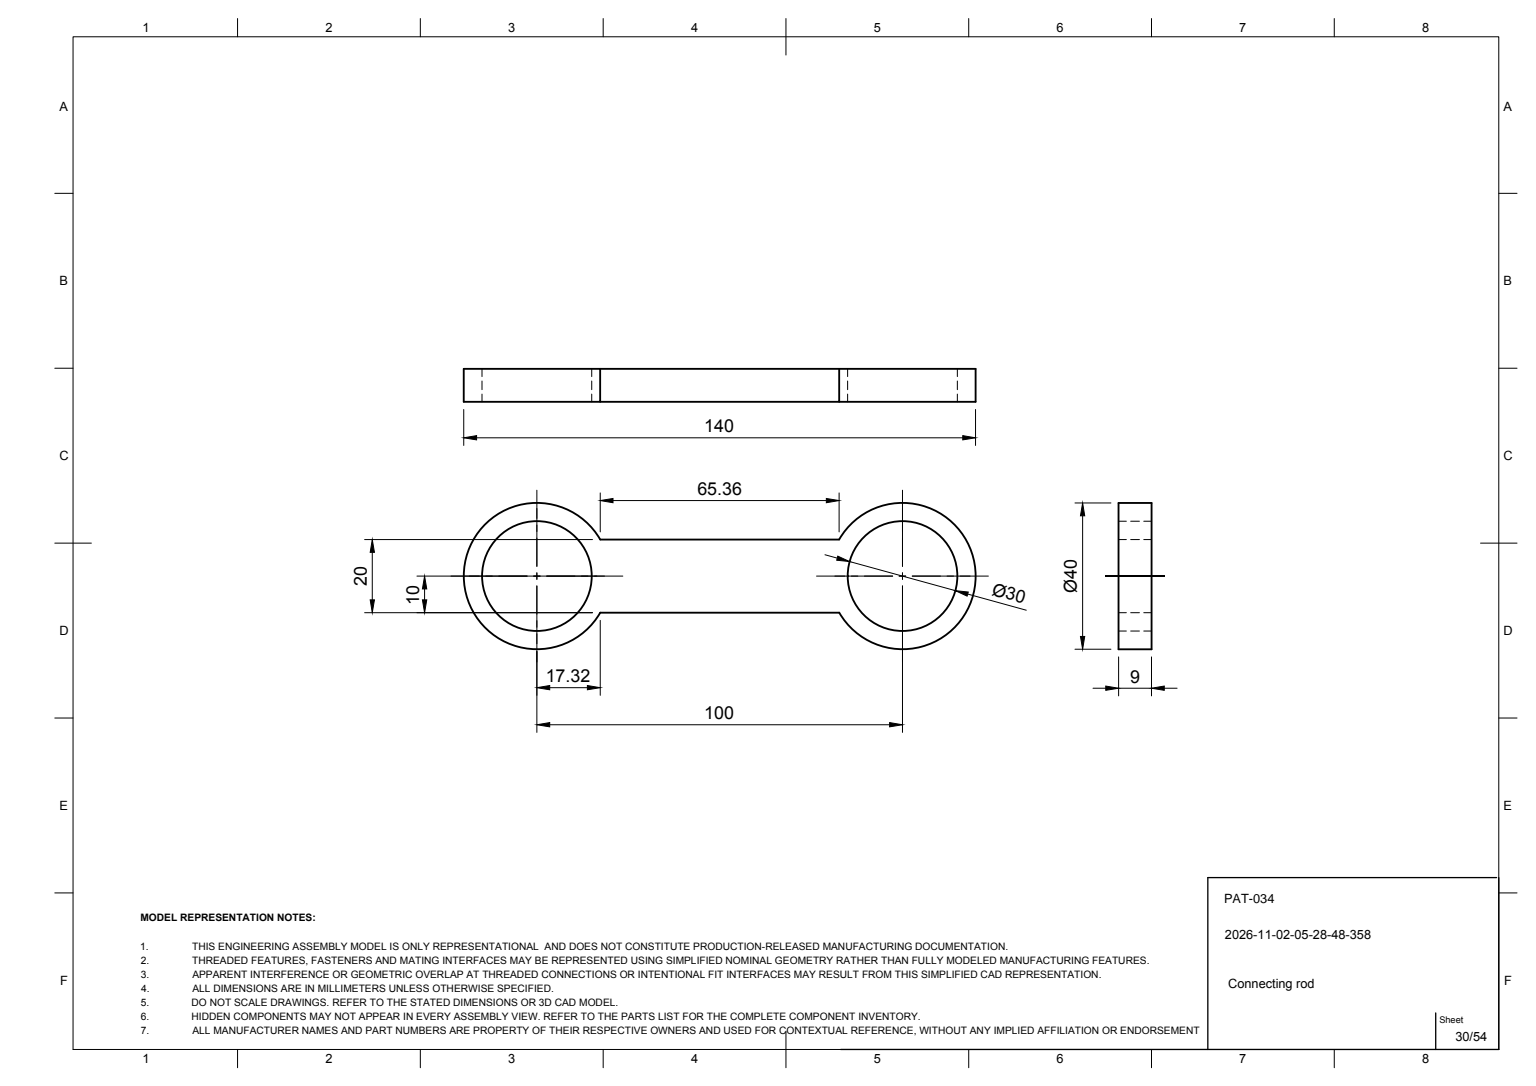
ISO-10303-21;
HEADER;
/* Generated by software containing ST-Developer
 * from STEP Tools, Inc. (www.steptools.com) 
 */

FILE_DESCRIPTION(
/* description */ ('Fatigue rig crank-slider'),
/* implementation_level */ '2;1');

FILE_NAME(
/* name */ 'Connecting rod.step',
/* time_stamp */ '2026-10-28T03:24:50-07:00',
/* author */ (''),
/* organization */ (''),
/* preprocessor_version */ 'ST-DEVELOPER v20.2',
/* originating_system */ 'Autodesk Translation Framework v15.17.0.0',
/* authorisation */ '');

FILE_SCHEMA (('AUTOMOTIVE_DESIGN { 1 0 10303 214 3 1 1 }'));
ENDSEC;

DATA;
#10=MECHANICAL_DESIGN_GEOMETRIC_PRESENTATION_REPRESENTATION('',(#615),#16911);
#514=SHAPE_REPRESENTATION_RELATIONSHIP('SRR','None',#17156,#564);
#564=ADVANCED_BREP_SHAPE_REPRESENTATION('',(#672),#16885);
#615=STYLED_ITEM('',(#17487),#672);
#672=MANIFOLD_SOLID_BREP('Body1',#8908);
#842=FACE_BOUND('',#2187,.T.);
#843=FACE_BOUND('',#2188,.T.);
#844=FACE_BOUND('',#2193,.T.);
#845=FACE_BOUND('',#2194,.T.);
#1082=PLANE('',#10063);
#1083=PLANE('',#10065);
#1084=PLANE('',#10068);
#1085=PLANE('',#10069);
#1518=FACE_OUTER_BOUND('',#2183,.T.);
#1519=FACE_OUTER_BOUND('',#2184,.T.);
#1520=FACE_OUTER_BOUND('',#2185,.T.);
#1521=FACE_OUTER_BOUND('',#2186,.T.);
#1522=FACE_OUTER_BOUND('',#2189,.T.);
#1523=FACE_OUTER_BOUND('',#2190,.T.);
#1524=FACE_OUTER_BOUND('',#2191,.T.);
#1525=FACE_OUTER_BOUND('',#2192,.T.);
#2183=EDGE_LOOP('',(#7256,#7257,#7258,#7259));
#2184=EDGE_LOOP('',(#7260,#7261,#7262,#7263));
#2185=EDGE_LOOP('',(#7264,#7265,#7266,#7267));
#2186=EDGE_LOOP('',(#7268,#7269,#7270,#7271));
#2187=EDGE_LOOP('',(#7272));
#2188=EDGE_LOOP('',(#7273));
#2189=EDGE_LOOP('',(#7274,#7275,#7276,#7277));
#2190=EDGE_LOOP('',(#7278,#7279,#7280,#7281));
#2191=EDGE_LOOP('',(#7282,#7283,#7284,#7285));
#2192=EDGE_LOOP('',(#7286,#7287,#7288,#7289));
#2193=EDGE_LOOP('',(#7290));
#2194=EDGE_LOOP('',(#7291));
#2829=LINE('',#15334,#3475);
#2830=LINE('',#15340,#3476);
#2831=LINE('',#15345,#3477);
#2832=LINE('',#15349,#3478);
#2833=LINE('',#15353,#3479);
#2834=LINE('',#15356,#3480);
#2835=LINE('',#15359,#3481);
#2836=LINE('',#15360,#3482);
#2837=LINE('',#15363,#3483);
#2838=LINE('',#15366,#3484);
#3475=VECTOR('',#12061,1.5);
#3476=VECTOR('',#12068,1.5);
#3477=VECTOR('',#12073,1.);
#3478=VECTOR('',#12076,1.);
#3479=VECTOR('',#12081,1.);
#3480=VECTOR('',#12084,1.);
#3481=VECTOR('',#12087,1.);
#3482=VECTOR('',#12088,1.);
#3483=VECTOR('',#12091,1.);
#3484=VECTOR('',#12096,1.);
#3977=CIRCLE('',#10055,1.5);
#3978=CIRCLE('',#10056,1.5);
#3979=CIRCLE('',#10058,1.5);
#3980=CIRCLE('',#10059,1.5);
#3981=CIRCLE('',#10061,2.);
#3982=CIRCLE('',#10062,2.);
#3983=CIRCLE('',#10064,2.);
#3984=CIRCLE('',#10067,2.);
#4577=VERTEX_POINT('',#15331);
#4578=VERTEX_POINT('',#15333);
#4579=VERTEX_POINT('',#15337);
#4580=VERTEX_POINT('',#15339);
#4581=VERTEX_POINT('',#15343);
#4582=VERTEX_POINT('',#15344);
#4583=VERTEX_POINT('',#15346);
#4584=VERTEX_POINT('',#15348);
#4585=VERTEX_POINT('',#15352);
#4586=VERTEX_POINT('',#15354);
#4587=VERTEX_POINT('',#15358);
#4588=VERTEX_POINT('',#15362);
#5526=EDGE_CURVE('',#4577,#4577,#3977,.T.);
#5527=EDGE_CURVE('',#4577,#4578,#2829,.T.);
#5528=EDGE_CURVE('',#4578,#4578,#3978,.T.);
#5529=EDGE_CURVE('',#4579,#4579,#3979,.T.);
#5530=EDGE_CURVE('',#4579,#4580,#2830,.T.);
#5531=EDGE_CURVE('',#4580,#4580,#3980,.T.);
#5532=EDGE_CURVE('',#4581,#4582,#2831,.T.);
#5533=EDGE_CURVE('',#4581,#4583,#3981,.T.);
#5534=EDGE_CURVE('',#4584,#4583,#2832,.T.);
#5535=EDGE_CURVE('',#4582,#4584,#3982,.T.);
#5536=EDGE_CURVE('',#4584,#4585,#2833,.T.);
#5537=EDGE_CURVE('',#4585,#4586,#3983,.T.);
#5538=EDGE_CURVE('',#4586,#4582,#2834,.T.);
#5539=EDGE_CURVE('',#4587,#4583,#2835,.T.);
#5540=EDGE_CURVE('',#4587,#4585,#2836,.T.);
#5541=EDGE_CURVE('',#4586,#4588,#2837,.T.);
#5542=EDGE_CURVE('',#4587,#4588,#3984,.T.);
#5543=EDGE_CURVE('',#4581,#4588,#2838,.T.);
#7256=ORIENTED_EDGE('',*,*,#5526,.F.);
#7257=ORIENTED_EDGE('',*,*,#5527,.T.);
#7258=ORIENTED_EDGE('',*,*,#5528,.F.);
#7259=ORIENTED_EDGE('',*,*,#5527,.F.);
#7260=ORIENTED_EDGE('',*,*,#5529,.F.);
#7261=ORIENTED_EDGE('',*,*,#5530,.T.);
#7262=ORIENTED_EDGE('',*,*,#5531,.F.);
#7263=ORIENTED_EDGE('',*,*,#5530,.F.);
#7264=ORIENTED_EDGE('',*,*,#5532,.F.);
#7265=ORIENTED_EDGE('',*,*,#5533,.T.);
#7266=ORIENTED_EDGE('',*,*,#5534,.F.);
#7267=ORIENTED_EDGE('',*,*,#5535,.F.);
#7268=ORIENTED_EDGE('',*,*,#5535,.T.);
#7269=ORIENTED_EDGE('',*,*,#5536,.T.);
#7270=ORIENTED_EDGE('',*,*,#5537,.T.);
#7271=ORIENTED_EDGE('',*,*,#5538,.T.);
#7272=ORIENTED_EDGE('',*,*,#5528,.T.);
#7273=ORIENTED_EDGE('',*,*,#5531,.T.);
#7274=ORIENTED_EDGE('',*,*,#5534,.T.);
#7275=ORIENTED_EDGE('',*,*,#5539,.F.);
#7276=ORIENTED_EDGE('',*,*,#5540,.T.);
#7277=ORIENTED_EDGE('',*,*,#5536,.F.);
#7278=ORIENTED_EDGE('',*,*,#5541,.F.);
#7279=ORIENTED_EDGE('',*,*,#5537,.F.);
#7280=ORIENTED_EDGE('',*,*,#5540,.F.);
#7281=ORIENTED_EDGE('',*,*,#5542,.T.);
#7282=ORIENTED_EDGE('',*,*,#5532,.T.);
#7283=ORIENTED_EDGE('',*,*,#5538,.F.);
#7284=ORIENTED_EDGE('',*,*,#5541,.T.);
#7285=ORIENTED_EDGE('',*,*,#5543,.F.);
#7286=ORIENTED_EDGE('',*,*,#5543,.T.);
#7287=ORIENTED_EDGE('',*,*,#5542,.F.);
#7288=ORIENTED_EDGE('',*,*,#5539,.T.);
#7289=ORIENTED_EDGE('',*,*,#5533,.F.);
#7290=ORIENTED_EDGE('',*,*,#5526,.T.);
#7291=ORIENTED_EDGE('',*,*,#5529,.T.);
#8301=CYLINDRICAL_SURFACE('',#10054,1.5);
#8302=CYLINDRICAL_SURFACE('',#10057,1.5);
#8303=CYLINDRICAL_SURFACE('',#10060,2.);
#8304=CYLINDRICAL_SURFACE('',#10066,2.);
#8656=ADVANCED_FACE('',(#1518),#8301,.F.);
#8657=ADVANCED_FACE('',(#1519),#8302,.F.);
#8658=ADVANCED_FACE('',(#1520),#8303,.T.);
#8659=ADVANCED_FACE('',(#1521,#842,#843),#1082,.T.);
#8660=ADVANCED_FACE('',(#1522),#1083,.T.);
#8661=ADVANCED_FACE('',(#1523),#8304,.T.);
#8662=ADVANCED_FACE('',(#1524),#1084,.T.);
#8663=ADVANCED_FACE('',(#1525,#844,#845),#1085,.F.);
#8908=CLOSED_SHELL('',(#8656,#8657,#8658,#8659,#8660,#8661,#8662,#8663));
#10053=AXIS2_PLACEMENT_3D('',#15329,#12055,#12056);
#10054=AXIS2_PLACEMENT_3D('',#15330,#12057,#12058);
#10055=AXIS2_PLACEMENT_3D('',#15332,#12059,#12060);
#10056=AXIS2_PLACEMENT_3D('',#15335,#12062,#12063);
#10057=AXIS2_PLACEMENT_3D('',#15336,#12064,#12065);
#10058=AXIS2_PLACEMENT_3D('',#15338,#12066,#12067);
#10059=AXIS2_PLACEMENT_3D('',#15341,#12069,#12070);
#10060=AXIS2_PLACEMENT_3D('',#15342,#12071,#12072);
#10061=AXIS2_PLACEMENT_3D('',#15347,#12074,#12075);
#10062=AXIS2_PLACEMENT_3D('',#15350,#12077,#12078);
#10063=AXIS2_PLACEMENT_3D('',#15351,#12079,#12080);
#10064=AXIS2_PLACEMENT_3D('',#15355,#12082,#12083);
#10065=AXIS2_PLACEMENT_3D('',#15357,#12085,#12086);
#10066=AXIS2_PLACEMENT_3D('',#15361,#12089,#12090);
#10067=AXIS2_PLACEMENT_3D('',#15364,#12092,#12093);
#10068=AXIS2_PLACEMENT_3D('',#15365,#12094,#12095);
#10069=AXIS2_PLACEMENT_3D('',#15367,#12097,#12098);
#12055=DIRECTION('axis',(0.,0.,1.));
#12056=DIRECTION('refdir',(1.,0.,0.));
#12057=DIRECTION('center_axis',(0.,1.,0.));
#12058=DIRECTION('ref_axis',(1.,0.,0.));
#12059=DIRECTION('center_axis',(0.,1.,0.));
#12060=DIRECTION('ref_axis',(1.,0.,0.));
#12061=DIRECTION('',(0.,1.,0.));
#12062=DIRECTION('center_axis',(0.,-1.,0.));
#12063=DIRECTION('ref_axis',(1.,0.,0.));
#12064=DIRECTION('center_axis',(0.,1.,0.));
#12065=DIRECTION('ref_axis',(1.,0.,0.));
#12066=DIRECTION('center_axis',(0.,1.,0.));
#12067=DIRECTION('ref_axis',(1.,0.,0.));
#12068=DIRECTION('',(0.,1.,0.));
#12069=DIRECTION('center_axis',(0.,-1.,0.));
#12070=DIRECTION('ref_axis',(1.,0.,0.));
#12071=DIRECTION('center_axis',(0.,1.,0.));
#12072=DIRECTION('ref_axis',(1.,0.,0.));
#12073=DIRECTION('',(0.,1.,0.));
#12074=DIRECTION('center_axis',(0.,1.,0.));
#12075=DIRECTION('ref_axis',(1.,0.,0.));
#12076=DIRECTION('',(0.,-1.,0.));
#12077=DIRECTION('center_axis',(0.,1.,0.));
#12078=DIRECTION('ref_axis',(1.,0.,0.));
#12079=DIRECTION('center_axis',(0.,1.,0.));
#12080=DIRECTION('ref_axis',(0.,0.,1.));
#12081=DIRECTION('',(-1.,0.,0.));
#12082=DIRECTION('center_axis',(0.,1.,0.));
#12083=DIRECTION('ref_axis',(1.,0.,0.));
#12084=DIRECTION('',(1.,0.,0.));
#12085=DIRECTION('center_axis',(0.,0.,-1.));
#12086=DIRECTION('ref_axis',(-1.,0.,0.));
#12087=DIRECTION('',(1.,0.,0.));
#12088=DIRECTION('',(0.,1.,0.));
#12089=DIRECTION('center_axis',(0.,1.,0.));
#12090=DIRECTION('ref_axis',(-1.,0.,1.22464679914735E-16));
#12091=DIRECTION('',(0.,-1.,0.));
#12092=DIRECTION('center_axis',(0.,1.,0.));
#12093=DIRECTION('ref_axis',(1.,0.,0.));
#12094=DIRECTION('center_axis',(0.,0.,1.));
#12095=DIRECTION('ref_axis',(1.,0.,0.));
#12096=DIRECTION('',(-1.,0.,0.));
#12097=DIRECTION('center_axis',(0.,1.,0.));
#12098=DIRECTION('ref_axis',(1.,0.,0.));
#15329=CARTESIAN_POINT('',(0.,0.,0.));
#15330=CARTESIAN_POINT('Origin',(1.,3.4,12.));
#15331=CARTESIAN_POINT('',(-0.5,3.5,12.));
#15332=CARTESIAN_POINT('Origin',(1.,3.5,12.));
#15333=CARTESIAN_POINT('',(-0.5,4.4,12.));
#15334=CARTESIAN_POINT('',(-0.5,3.4,12.));
#15335=CARTESIAN_POINT('Origin',(1.,4.4,12.));
#15336=CARTESIAN_POINT('Origin',(11.,3.4,12.));
#15337=CARTESIAN_POINT('',(9.5,3.5,12.));
#15338=CARTESIAN_POINT('Origin',(11.,3.5,12.));
#15339=CARTESIAN_POINT('',(9.5,4.4,12.));
#15340=CARTESIAN_POINT('',(9.5,3.4,12.));
#15341=CARTESIAN_POINT('Origin',(11.,4.4,12.));
#15342=CARTESIAN_POINT('Origin',(11.,3.5,12.));
#15343=CARTESIAN_POINT('',(9.26794919243112,3.5,13.));
#15344=CARTESIAN_POINT('',(9.26794919243112,4.4,13.));
#15345=CARTESIAN_POINT('',(9.26794919243112,3.5,13.));
#15346=CARTESIAN_POINT('',(9.26794919243112,3.5,11.));
#15347=CARTESIAN_POINT('Origin',(11.,3.5,12.));
#15348=CARTESIAN_POINT('',(9.26794919243112,4.4,11.));
#15349=CARTESIAN_POINT('',(9.26794919243112,3.5,11.));
#15350=CARTESIAN_POINT('Origin',(11.,4.4,12.));
#15351=CARTESIAN_POINT('Origin',(6.,4.4,12.));
#15352=CARTESIAN_POINT('',(2.73205080756888,4.4,11.));
#15353=CARTESIAN_POINT('',(1.,4.4,11.));
#15354=CARTESIAN_POINT('',(2.73205080756888,4.4,13.));
#15355=CARTESIAN_POINT('Origin',(1.,4.4,12.));
#15356=CARTESIAN_POINT('',(11.,4.4,13.));
#15357=CARTESIAN_POINT('Origin',(11.,3.5,11.));
#15358=CARTESIAN_POINT('',(2.73205080756888,3.5,11.));
#15359=CARTESIAN_POINT('',(1.,3.5,11.));
#15360=CARTESIAN_POINT('',(2.73205080756888,3.5,11.));
#15361=CARTESIAN_POINT('Origin',(1.,3.5,12.));
#15362=CARTESIAN_POINT('',(2.73205080756888,3.5,13.));
#15363=CARTESIAN_POINT('',(2.73205080756888,3.5,13.));
#15364=CARTESIAN_POINT('Origin',(1.,3.5,12.));
#15365=CARTESIAN_POINT('Origin',(1.,3.5,13.));
#15366=CARTESIAN_POINT('',(11.,3.5,13.));
#15367=CARTESIAN_POINT('Origin',(6.,3.5,12.));
#16826=UNCERTAINTY_MEASURE_WITH_UNIT(LENGTH_MEASURE(0.001),#16912,
'DISTANCE_ACCURACY_VALUE',
'Maximum model space distance between geometric entities at asserted c
onnectivities');
#16852=UNCERTAINTY_MEASURE_WITH_UNIT(LENGTH_MEASURE(0.001),#16912,
'DISTANCE_ACCURACY_VALUE',
'Maximum model space distance between geometric entities at asserted c
onnectivities');
#16885=(
GEOMETRIC_REPRESENTATION_CONTEXT(3)
GLOBAL_UNCERTAINTY_ASSIGNED_CONTEXT((#16826))
GLOBAL_UNIT_ASSIGNED_CONTEXT((#16912,#16914,#16915))
REPRESENTATION_CONTEXT('','3D')
);
#16911=(
GEOMETRIC_REPRESENTATION_CONTEXT(3)
GLOBAL_UNCERTAINTY_ASSIGNED_CONTEXT((#16852))
GLOBAL_UNIT_ASSIGNED_CONTEXT((#16912,#16914,#16915))
REPRESENTATION_CONTEXT('','3D')
);
#16912=(
LENGTH_UNIT()
NAMED_UNIT(*)
SI_UNIT(.CENTI.,.METRE.)
);
#16914=(
NAMED_UNIT(*)
PLANE_ANGLE_UNIT()
SI_UNIT($,.RADIAN.)
);
#16915=(
NAMED_UNIT(*)
SI_UNIT($,.STERADIAN.)
SOLID_ANGLE_UNIT()
);
#16948=SHAPE_DEFINITION_REPRESENTATION(#17008,#17156);
#17008=PRODUCT_DEFINITION_SHAPE('',$,#17215);
#17156=SHAPE_REPRESENTATION('',(#10053),#16885);
#17182=PRODUCT_DEFINITION_CONTEXT('part definition',#17358,'design');
#17215=PRODUCT_DEFINITION('Connecting rod','Connecting rod',#17273,#17182);
#17273=PRODUCT_DEFINITION_FORMATION('',$,#17392);
#17358=APPLICATION_CONTEXT(
'Core Data for Automotive Mechanical Design Process');
#17359=PRODUCT_CONTEXT('part definition',#17358,'mechanical');
#17392=PRODUCT('Connecting rod','Connecting rod','Connecting rod',(#17359));
#17481=COLOUR_RGB('Grey',0.48,0.52,0.57);
#17482=FILL_AREA_STYLE_COLOUR('',#17481);
#17483=FILL_AREA_STYLE('',(#17482));
#17484=SURFACE_STYLE_FILL_AREA(#17483);
#17485=SURFACE_SIDE_STYLE('',(#17484));
#17486=SURFACE_STYLE_USAGE(.BOTH.,#17485);
#17487=PRESENTATION_STYLE_ASSIGNMENT((#17486));
ENDSEC;
END-ISO-10303-21;
